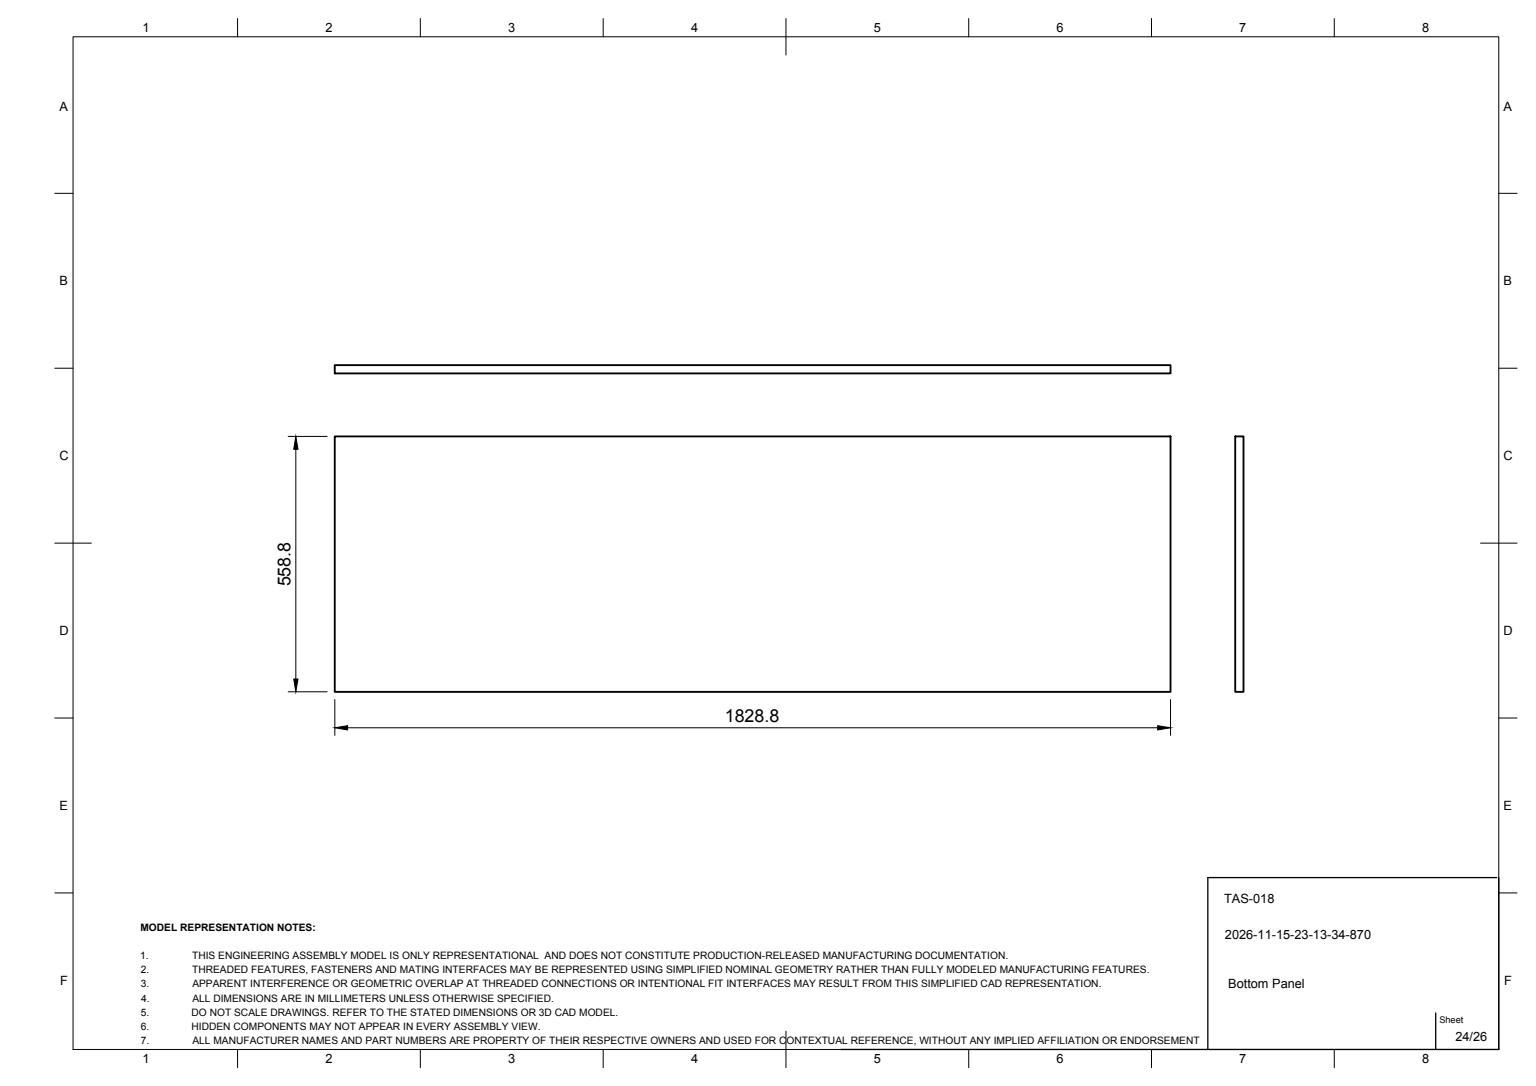
ISO-10303-21;
HEADER;
/* Generated by software containing ST-Developer
 * from STEP Tools, Inc. (www.steptools.com) 
 */

FILE_DESCRIPTION(
/* description */ (''),
/* implementation_level */ '2;1');

FILE_NAME(
/* name */ 'Bottom Panel.step',
/* time_stamp */ '2026-11-15T15:17:57-08:00',
/* author */ (''),
/* organization */ (''),
/* preprocessor_version */ 'ST-DEVELOPER v20.2',
/* originating_system */ 'Autodesk Translation Framework v15.17.0.0',
/* authorisation */ '');

FILE_SCHEMA (('AUTOMOTIVE_DESIGN { 1 0 10303 214 3 1 1 }'));
ENDSEC;

DATA;
#10=MECHANICAL_DESIGN_GEOMETRIC_PRESENTATION_REPRESENTATION('',(#199),#3723);
#151=SHAPE_REPRESENTATION_RELATIONSHIP('SRR','None',#3832,#175);
#175=ADVANCED_BREP_SHAPE_REPRESENTATION('',(#223),#3721);
#199=STYLED_ITEM('',(#3948),#223);
#223=MANIFOLD_SOLID_BREP('Body1',#2047);
#339=FACE_OUTER_BOUND('',#465,.T.);
#340=FACE_OUTER_BOUND('',#466,.T.);
#341=FACE_OUTER_BOUND('',#467,.T.);
#342=FACE_OUTER_BOUND('',#468,.T.);
#343=FACE_OUTER_BOUND('',#469,.T.);
#344=FACE_OUTER_BOUND('',#470,.T.);
#465=EDGE_LOOP('',(#1731,#1732,#1733,#1734));
#466=EDGE_LOOP('',(#1735,#1736,#1737,#1738));
#467=EDGE_LOOP('',(#1739,#1740,#1741,#1742));
#468=EDGE_LOOP('',(#1743,#1744,#1745,#1746));
#469=EDGE_LOOP('',(#1747,#1748,#1749,#1750));
#470=EDGE_LOOP('',(#1751,#1752,#1753,#1754));
#675=LINE('',#3596,#897);
#676=LINE('',#3598,#898);
#677=LINE('',#3600,#899);
#678=LINE('',#3601,#900);
#679=LINE('',#3604,#901);
#680=LINE('',#3606,#902);
#681=LINE('',#3607,#903);
#682=LINE('',#3610,#904);
#683=LINE('',#3612,#905);
#684=LINE('',#3613,#906);
#685=LINE('',#3615,#907);
#686=LINE('',#3616,#908);
#897=VECTOR('',#3007,22.);
#898=VECTOR('',#3008,0.708661417322835);
#899=VECTOR('',#3009,22.);
#900=VECTOR('',#3010,0.708661417322835);
#901=VECTOR('',#3013,72.);
#902=VECTOR('',#3014,0.708661417322835);
#903=VECTOR('',#3015,72.);
#904=VECTOR('',#3018,22.);
#905=VECTOR('',#3019,0.708661417322835);
#906=VECTOR('',#3020,22.);
#907=VECTOR('',#3023,72.);
#908=VECTOR('',#3024,72.);
#1061=VERTEX_POINT('',#3594);
#1062=VERTEX_POINT('',#3595);
#1063=VERTEX_POINT('',#3597);
#1064=VERTEX_POINT('',#3599);
#1065=VERTEX_POINT('',#3603);
#1066=VERTEX_POINT('',#3605);
#1067=VERTEX_POINT('',#3609);
#1068=VERTEX_POINT('',#3611);
#1287=EDGE_CURVE('',#1061,#1062,#675,.T.);
#1288=EDGE_CURVE('',#1063,#1062,#676,.T.);
#1289=EDGE_CURVE('',#1064,#1063,#677,.T.);
#1290=EDGE_CURVE('',#1064,#1061,#678,.T.);
#1291=EDGE_CURVE('',#1062,#1065,#679,.T.);
#1292=EDGE_CURVE('',#1066,#1065,#680,.T.);
#1293=EDGE_CURVE('',#1063,#1066,#681,.T.);
#1294=EDGE_CURVE('',#1065,#1067,#682,.T.);
#1295=EDGE_CURVE('',#1068,#1067,#683,.T.);
#1296=EDGE_CURVE('',#1066,#1068,#684,.T.);
#1297=EDGE_CURVE('',#1067,#1061,#685,.T.);
#1298=EDGE_CURVE('',#1068,#1064,#686,.T.);
#1731=ORIENTED_EDGE('',*,*,#1287,.T.);
#1732=ORIENTED_EDGE('',*,*,#1288,.F.);
#1733=ORIENTED_EDGE('',*,*,#1289,.F.);
#1734=ORIENTED_EDGE('',*,*,#1290,.T.);
#1735=ORIENTED_EDGE('',*,*,#1291,.T.);
#1736=ORIENTED_EDGE('',*,*,#1292,.F.);
#1737=ORIENTED_EDGE('',*,*,#1293,.F.);
#1738=ORIENTED_EDGE('',*,*,#1288,.T.);
#1739=ORIENTED_EDGE('',*,*,#1294,.T.);
#1740=ORIENTED_EDGE('',*,*,#1295,.F.);
#1741=ORIENTED_EDGE('',*,*,#1296,.F.);
#1742=ORIENTED_EDGE('',*,*,#1292,.T.);
#1743=ORIENTED_EDGE('',*,*,#1297,.T.);
#1744=ORIENTED_EDGE('',*,*,#1290,.F.);
#1745=ORIENTED_EDGE('',*,*,#1298,.F.);
#1746=ORIENTED_EDGE('',*,*,#1295,.T.);
#1747=ORIENTED_EDGE('',*,*,#1289,.T.);
#1748=ORIENTED_EDGE('',*,*,#1293,.T.);
#1749=ORIENTED_EDGE('',*,*,#1296,.T.);
#1750=ORIENTED_EDGE('',*,*,#1298,.T.);
#1751=ORIENTED_EDGE('',*,*,#1287,.F.);
#1752=ORIENTED_EDGE('',*,*,#1297,.F.);
#1753=ORIENTED_EDGE('',*,*,#1294,.F.);
#1754=ORIENTED_EDGE('',*,*,#1291,.F.);
#1887=PLANE('',#2466);
#1888=PLANE('',#2467);
#1889=PLANE('',#2468);
#1890=PLANE('',#2469);
#1891=PLANE('',#2470);
#1892=PLANE('',#2471);
#2013=ADVANCED_FACE('',(#339),#1887,.F.);
#2014=ADVANCED_FACE('',(#340),#1888,.F.);
#2015=ADVANCED_FACE('',(#341),#1889,.F.);
#2016=ADVANCED_FACE('',(#342),#1890,.F.);
#2017=ADVANCED_FACE('',(#343),#1891,.T.);
#2018=ADVANCED_FACE('',(#344),#1892,.F.);
#2047=CLOSED_SHELL('',(#2013,#2014,#2015,#2016,#2017,#2018));
#2465=AXIS2_PLACEMENT_3D('',#3592,#3003,#3004);
#2466=AXIS2_PLACEMENT_3D('',#3593,#3005,#3006);
#2467=AXIS2_PLACEMENT_3D('',#3602,#3011,#3012);
#2468=AXIS2_PLACEMENT_3D('',#3608,#3016,#3017);
#2469=AXIS2_PLACEMENT_3D('',#3614,#3021,#3022);
#2470=AXIS2_PLACEMENT_3D('',#3617,#3025,#3026);
#2471=AXIS2_PLACEMENT_3D('',#3618,#3027,#3028);
#3003=DIRECTION('axis',(0.,0.,1.));
#3004=DIRECTION('refdir',(1.,0.,0.));
#3005=DIRECTION('center_axis',(1.,0.,1.98679854084674E-16));
#3006=DIRECTION('ref_axis',(1.98679854084674E-16,0.,-1.));
#3007=DIRECTION('',(2.54310213228382E-16,0.,-1.));
#3008=DIRECTION('',(0.,1.,0.));
#3009=DIRECTION('',(2.54310213228382E-16,0.,-1.));
#3010=DIRECTION('',(0.,1.,0.));
#3011=DIRECTION('center_axis',(0.,0.,1.));
#3012=DIRECTION('ref_axis',(1.,0.,0.));
#3013=DIRECTION('',(1.,0.,0.));
#3014=DIRECTION('',(0.,1.,0.));
#3015=DIRECTION('',(1.,0.,0.));
#3016=DIRECTION('center_axis',(-1.,0.,-3.97359708169347E-16));
#3017=DIRECTION('ref_axis',(-3.97359708169347E-16,0.,1.));
#3018=DIRECTION('',(-2.54310213228382E-16,0.,1.));
#3019=DIRECTION('',(0.,1.,0.));
#3020=DIRECTION('',(-2.54310213228382E-16,0.,1.));
#3021=DIRECTION('center_axis',(0.,0.,-1.));
#3022=DIRECTION('ref_axis',(-1.,0.,0.));
#3023=DIRECTION('',(-1.,0.,0.));
#3024=DIRECTION('',(-1.,0.,0.));
#3025=DIRECTION('center_axis',(0.,-1.,0.));
#3026=DIRECTION('ref_axis',(0.,0.,-1.));
#3027=DIRECTION('center_axis',(0.,-1.,0.));
#3028=DIRECTION('ref_axis',(0.,0.,-1.));
#3592=CARTESIAN_POINT('',(0.,0.,0.));
#3593=CARTESIAN_POINT('Origin',(-36.,3.93700787401574,22.));
#3594=CARTESIAN_POINT('',(-36.,4.64566929133858,22.));
#3595=CARTESIAN_POINT('',(-36.,4.64566929133858,0.));
#3596=CARTESIAN_POINT('',(-36.,4.64566929133858,22.));
#3597=CARTESIAN_POINT('',(-36.,3.93700787401574,0.));
#3598=CARTESIAN_POINT('',(-36.,3.93700787401574,0.));
#3599=CARTESIAN_POINT('',(-36.,3.93700787401574,22.));
#3600=CARTESIAN_POINT('',(-36.,3.93700787401574,22.));
#3601=CARTESIAN_POINT('',(-36.,3.93700787401574,22.));
#3602=CARTESIAN_POINT('Origin',(-36.,3.93700787401574,0.));
#3603=CARTESIAN_POINT('',(36.,4.64566929133858,0.));
#3604=CARTESIAN_POINT('',(-36.,4.64566929133858,0.));
#3605=CARTESIAN_POINT('',(36.,3.93700787401574,0.));
#3606=CARTESIAN_POINT('',(36.,3.93700787401574,0.));
#3607=CARTESIAN_POINT('',(-36.,3.93700787401574,0.));
#3608=CARTESIAN_POINT('Origin',(36.,3.93700787401574,22.));
#3609=CARTESIAN_POINT('',(36.,4.64566929133858,22.));
#3610=CARTESIAN_POINT('',(36.,4.64566929133858,0.));
#3611=CARTESIAN_POINT('',(36.,3.93700787401574,22.));
#3612=CARTESIAN_POINT('',(36.,3.93700787401574,22.));
#3613=CARTESIAN_POINT('',(36.,3.93700787401574,0.));
#3614=CARTESIAN_POINT('Origin',(-36.,3.93700787401574,22.));
#3615=CARTESIAN_POINT('',(36.,4.64566929133858,22.));
#3616=CARTESIAN_POINT('',(36.,3.93700787401574,22.));
#3617=CARTESIAN_POINT('Origin',(0.,3.93700787401574,0.));
#3618=CARTESIAN_POINT('Origin',(0.,4.64566929133858,0.));
#3694=UNCERTAINTY_MEASURE_WITH_UNIT(LENGTH_MEASURE(0.000393700787401575),
#3725,'DISTANCE_ACCURACY_VALUE',
'Maximum model space distance between geometric entities at asserted c
onnectivities');
#3696=UNCERTAINTY_MEASURE_WITH_UNIT(LENGTH_MEASURE(0.000393700787401575),
#3725,'DISTANCE_ACCURACY_VALUE',
'Maximum model space distance between geometric entities at asserted c
onnectivities');
#3721=(
GEOMETRIC_REPRESENTATION_CONTEXT(3)
GLOBAL_UNCERTAINTY_ASSIGNED_CONTEXT((#3694))
GLOBAL_UNIT_ASSIGNED_CONTEXT((#3725,#3729,#3730))
REPRESENTATION_CONTEXT('','3D')
);
#3723=(
GEOMETRIC_REPRESENTATION_CONTEXT(3)
GLOBAL_UNCERTAINTY_ASSIGNED_CONTEXT((#3696))
GLOBAL_UNIT_ASSIGNED_CONTEXT((#3725,#3729,#3730))
REPRESENTATION_CONTEXT('','3D')
);
#3724=DIMENSIONAL_EXPONENTS(1.,0.,0.,0.,0.,0.,0.);
#3725=(
CONVERSION_BASED_UNIT('inch',#3728)
LENGTH_UNIT()
NAMED_UNIT(#3724)
);
#3726=(
LENGTH_UNIT()
NAMED_UNIT(*)
SI_UNIT(.MILLI.,.METRE.)
);
#3728=LENGTH_MEASURE_WITH_UNIT(LENGTH_MEASURE(25.4),#3726);
#3729=(
NAMED_UNIT(*)
PLANE_ANGLE_UNIT()
SI_UNIT($,.RADIAN.)
);
#3730=(
NAMED_UNIT(*)
SI_UNIT($,.STERADIAN.)
SOLID_ANGLE_UNIT()
);
#3755=SHAPE_DEFINITION_REPRESENTATION(#3782,#3832);
#3782=PRODUCT_DEFINITION_SHAPE('',$,#3859);
#3832=SHAPE_REPRESENTATION('',(#2465),#3721);
#3834=PRODUCT_DEFINITION_CONTEXT('part definition',#3914,'design');
#3859=PRODUCT_DEFINITION('2026-11-15-23-13-34-870','Bottom Panel',#3885,
#3834);
#3885=PRODUCT_DEFINITION_FORMATION('',$,#3940);
#3914=APPLICATION_CONTEXT(
'Core Data for Automotive Mechanical Design Process');
#3915=PRODUCT_CONTEXT('part definition',#3914,'mechanical');
#3940=PRODUCT('2026-11-15-23-13-34-870','Bottom Panel',$,(#3915));
#3948=PRESENTATION_STYLE_ASSIGNMENT((#3956));
#3956=SURFACE_STYLE_USAGE(.BOTH.,#3964);
#3964=SURFACE_SIDE_STYLE('',(#3972));
#3972=SURFACE_STYLE_FILL_AREA(#3980);
#3980=FILL_AREA_STYLE('Blue',(#3988));
#3988=FILL_AREA_STYLE_COLOUR('Blue',#3996);
#3996=COLOUR_RGB('Blue',0.,0.4,0.8);
ENDSEC;
END-ISO-10303-21;
